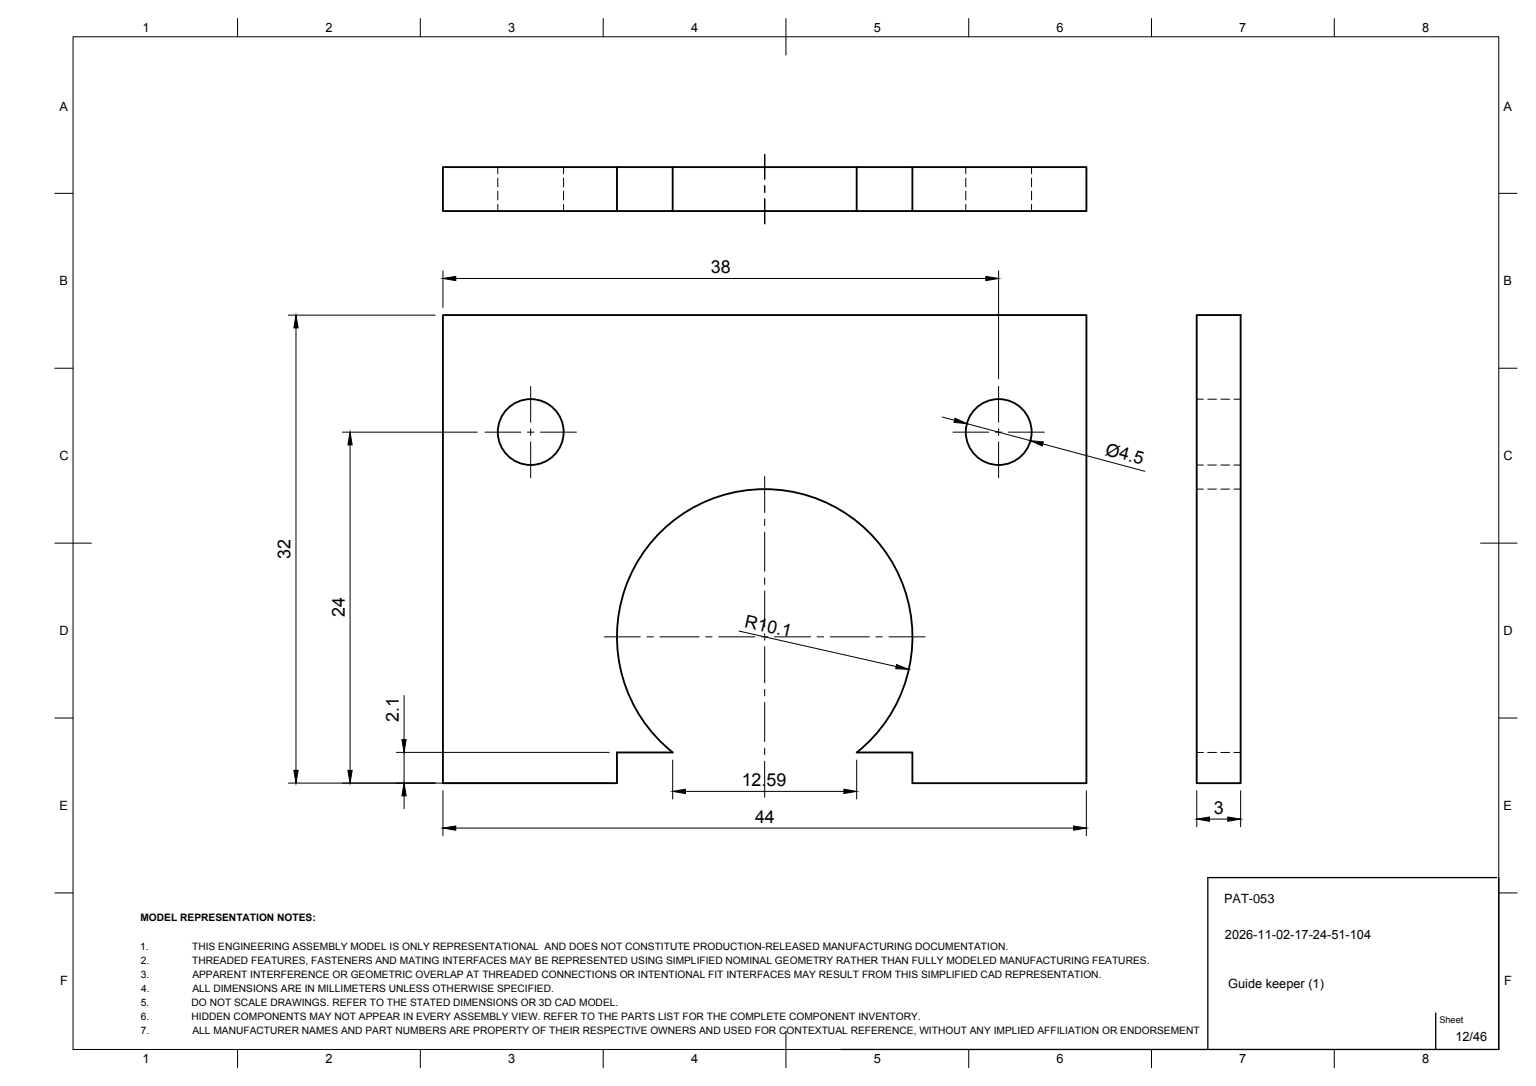
ISO-10303-21;
HEADER;
/* Generated by software containing ST-Developer
 * from STEP Tools, Inc. (www.steptools.com) 
 */

FILE_DESCRIPTION(
/* description */ ('Hand-operated arbor press'),
/* implementation_level */ '2;1');

FILE_NAME(
/* name */ 'Guide keeper (1).step',
/* time_stamp */ '2026-10-28T03:25:25-07:00',
/* author */ (''),
/* organization */ (''),
/* preprocessor_version */ 'ST-DEVELOPER v20.2',
/* originating_system */ 'Autodesk Translation Framework v15.17.0.0',
/* authorisation */ '');

FILE_SCHEMA (('AUTOMOTIVE_DESIGN { 1 0 10303 214 3 1 1 }'));
ENDSEC;

DATA;
#10=MECHANICAL_DESIGN_GEOMETRIC_PRESENTATION_REPRESENTATION('',(#593),#32751);
#509=SHAPE_REPRESENTATION_RELATIONSHIP('SRR','None',#32938,#551);
#551=ADVANCED_BREP_SHAPE_REPRESENTATION('',(#642),#32712);
#593=STYLED_ITEM('',(#33235),#642);
#642=MANIFOLD_SOLID_BREP('Body1',#12490);
#719=FACE_BOUND('',#2125,.T.);
#720=FACE_BOUND('',#2126,.T.);
#721=FACE_BOUND('',#2132,.T.);
#722=FACE_BOUND('',#2133,.T.);
#919=PLANE('',#13184);
#920=PLANE('',#13185);
#921=PLANE('',#13186);
#922=PLANE('',#13187);
#923=PLANE('',#13188);
#924=PLANE('',#13189);
#925=PLANE('',#13190);
#926=PLANE('',#13194);
#927=PLANE('',#13195);
#928=PLANE('',#13196);
#929=PLANE('',#13197);
#1396=FACE_OUTER_BOUND('',#2116,.T.);
#1397=FACE_OUTER_BOUND('',#2117,.T.);
#1398=FACE_OUTER_BOUND('',#2118,.T.);
#1399=FACE_OUTER_BOUND('',#2119,.T.);
#1400=FACE_OUTER_BOUND('',#2120,.T.);
#1401=FACE_OUTER_BOUND('',#2121,.T.);
#1402=FACE_OUTER_BOUND('',#2122,.T.);
#1403=FACE_OUTER_BOUND('',#2123,.T.);
#1404=FACE_OUTER_BOUND('',#2124,.T.);
#1405=FACE_OUTER_BOUND('',#2127,.T.);
#1406=FACE_OUTER_BOUND('',#2128,.T.);
#1407=FACE_OUTER_BOUND('',#2129,.T.);
#1408=FACE_OUTER_BOUND('',#2130,.T.);
#1409=FACE_OUTER_BOUND('',#2131,.T.);
#2116=EDGE_LOOP('',(#8816,#8817,#8818,#8819));
#2117=EDGE_LOOP('',(#8820,#8821,#8822,#8823));
#2118=EDGE_LOOP('',(#8824,#8825,#8826,#8827));
#2119=EDGE_LOOP('',(#8828,#8829,#8830,#8831));
#2120=EDGE_LOOP('',(#8832,#8833,#8834,#8835));
#2121=EDGE_LOOP('',(#8836,#8837,#8838,#8839));
#2122=EDGE_LOOP('',(#8840,#8841,#8842,#8843));
#2123=EDGE_LOOP('',(#8844,#8845,#8846,#8847));
#2124=EDGE_LOOP('',(#8848,#8849,#8850,#8851,#8852,#8853,#8854,#8855,#8856,
#8857));
#2125=EDGE_LOOP('',(#8858));
#2126=EDGE_LOOP('',(#8859));
#2127=EDGE_LOOP('',(#8860,#8861,#8862,#8863));
#2128=EDGE_LOOP('',(#8864,#8865,#8866,#8867));
#2129=EDGE_LOOP('',(#8868,#8869,#8870,#8871));
#2130=EDGE_LOOP('',(#8872,#8873,#8874,#8875));
#2131=EDGE_LOOP('',(#8876,#8877,#8878,#8879,#8880,#8881,#8882,#8883,#8884,
#8885));
#2132=EDGE_LOOP('',(#8886));
#2133=EDGE_LOOP('',(#8887));
#3004=LINE('',#18165,#4175);
#3005=LINE('',#18171,#4176);
#3006=LINE('',#18176,#4177);
#3007=LINE('',#18178,#4178);
#3008=LINE('',#18180,#4179);
#3009=LINE('',#18181,#4180);
#3010=LINE('',#18185,#4181);
#3011=LINE('',#18187,#4182);
#3012=LINE('',#18189,#4183);
#3013=LINE('',#18190,#4184);
#3014=LINE('',#18193,#4185);
#3015=LINE('',#18195,#4186);
#3016=LINE('',#18196,#4187);
#3017=LINE('',#18199,#4188);
#3018=LINE('',#18201,#4189);
#3019=LINE('',#18202,#4190);
#3020=LINE('',#18205,#4191);
#3021=LINE('',#18207,#4192);
#3022=LINE('',#18208,#4193);
#3023=LINE('',#18211,#4194);
#3024=LINE('',#18213,#4195);
#3025=LINE('',#18214,#4196);
#3026=LINE('',#18218,#4197);
#3027=LINE('',#18220,#4198);
#3028=LINE('',#18221,#4199);
#3029=LINE('',#18226,#4200);
#3030=LINE('',#18227,#4201);
#3031=LINE('',#18230,#4202);
#3032=LINE('',#18231,#4203);
#3033=LINE('',#18233,#4204);
#4175=VECTOR('',#14697,0.225);
#4176=VECTOR('',#14704,0.225);
#4177=VECTOR('',#14709,1.);
#4178=VECTOR('',#14710,1.);
#4179=VECTOR('',#14711,1.);
#4180=VECTOR('',#14712,1.);
#4181=VECTOR('',#14715,1.);
#4182=VECTOR('',#14716,1.);
#4183=VECTOR('',#14717,1.);
#4184=VECTOR('',#14718,1.);
#4185=VECTOR('',#14721,1.);
#4186=VECTOR('',#14722,1.);
#4187=VECTOR('',#14723,1.);
#4188=VECTOR('',#14726,1.);
#4189=VECTOR('',#14727,1.);
#4190=VECTOR('',#14728,1.);
#4191=VECTOR('',#14731,1.);
#4192=VECTOR('',#14732,1.);
#4193=VECTOR('',#14733,1.);
#4194=VECTOR('',#14736,1.);
#4195=VECTOR('',#14737,1.);
#4196=VECTOR('',#14738,1.);
#4197=VECTOR('',#14743,1.);
#4198=VECTOR('',#14744,1.);
#4199=VECTOR('',#14745,1.);
#4200=VECTOR('',#14752,1.);
#4201=VECTOR('',#14753,1.);
#4202=VECTOR('',#14756,1.);
#4203=VECTOR('',#14757,1.);
#4204=VECTOR('',#14760,1.);
#5232=CIRCLE('',#13179,0.225);
#5233=CIRCLE('',#13180,0.225);
#5234=CIRCLE('',#13182,0.225);
#5235=CIRCLE('',#13183,0.225);
#5236=CIRCLE('',#13191,1.01);
#5237=CIRCLE('',#13193,1.01);
#5720=VERTEX_POINT('',#18162);
#5721=VERTEX_POINT('',#18164);
#5722=VERTEX_POINT('',#18168);
#5723=VERTEX_POINT('',#18170);
#5724=VERTEX_POINT('',#18174);
#5725=VERTEX_POINT('',#18175);
#5726=VERTEX_POINT('',#18177);
#5727=VERTEX_POINT('',#18179);
#5728=VERTEX_POINT('',#18183);
#5729=VERTEX_POINT('',#18184);
#5730=VERTEX_POINT('',#18186);
#5731=VERTEX_POINT('',#18188);
#5732=VERTEX_POINT('',#18192);
#5733=VERTEX_POINT('',#18194);
#5734=VERTEX_POINT('',#18198);
#5735=VERTEX_POINT('',#18200);
#5736=VERTEX_POINT('',#18204);
#5737=VERTEX_POINT('',#18206);
#5738=VERTEX_POINT('',#18210);
#5739=VERTEX_POINT('',#18212);
#5740=VERTEX_POINT('',#18217);
#5741=VERTEX_POINT('',#18219);
#5742=VERTEX_POINT('',#18225);
#5743=VERTEX_POINT('',#18229);
#6911=EDGE_CURVE('',#5720,#5720,#5232,.T.);
#6912=EDGE_CURVE('',#5720,#5721,#3004,.T.);
#6913=EDGE_CURVE('',#5721,#5721,#5233,.T.);
#6914=EDGE_CURVE('',#5722,#5722,#5234,.T.);
#6915=EDGE_CURVE('',#5722,#5723,#3005,.T.);
#6916=EDGE_CURVE('',#5723,#5723,#5235,.T.);
#6917=EDGE_CURVE('',#5724,#5725,#3006,.T.);
#6918=EDGE_CURVE('',#5724,#5726,#3007,.T.);
#6919=EDGE_CURVE('',#5727,#5726,#3008,.T.);
#6920=EDGE_CURVE('',#5725,#5727,#3009,.T.);
#6921=EDGE_CURVE('',#5728,#5729,#3010,.T.);
#6922=EDGE_CURVE('',#5730,#5728,#3011,.T.);
#6923=EDGE_CURVE('',#5731,#5730,#3012,.T.);
#6924=EDGE_CURVE('',#5729,#5731,#3013,.T.);
#6925=EDGE_CURVE('',#5732,#5728,#3014,.T.);
#6926=EDGE_CURVE('',#5733,#5732,#3015,.T.);
#6927=EDGE_CURVE('',#5730,#5733,#3016,.T.);
#6928=EDGE_CURVE('',#5734,#5724,#3017,.T.);
#6929=EDGE_CURVE('',#5735,#5734,#3018,.T.);
#6930=EDGE_CURVE('',#5726,#5735,#3019,.T.);
#6931=EDGE_CURVE('',#5736,#5727,#3020,.T.);
#6932=EDGE_CURVE('',#5737,#5736,#3021,.T.);
#6933=EDGE_CURVE('',#5737,#5725,#3022,.T.);
#6934=EDGE_CURVE('',#5731,#5738,#3023,.T.);
#6935=EDGE_CURVE('',#5738,#5739,#3024,.T.);
#6936=EDGE_CURVE('',#5729,#5739,#3025,.T.);
#6937=EDGE_CURVE('',#5735,#5732,#5236,.T.);
#6938=EDGE_CURVE('',#5739,#5740,#3026,.T.);
#6939=EDGE_CURVE('',#5740,#5741,#3027,.T.);
#6940=EDGE_CURVE('',#5741,#5736,#3028,.T.);
#6941=EDGE_CURVE('',#5733,#5734,#5237,.T.);
#6942=EDGE_CURVE('',#5742,#5737,#3029,.T.);
#6943=EDGE_CURVE('',#5742,#5741,#3030,.T.);
#6944=EDGE_CURVE('',#5743,#5742,#3031,.T.);
#6945=EDGE_CURVE('',#5743,#5740,#3032,.T.);
#6946=EDGE_CURVE('',#5738,#5743,#3033,.T.);
#8816=ORIENTED_EDGE('',*,*,#6911,.F.);
#8817=ORIENTED_EDGE('',*,*,#6912,.T.);
#8818=ORIENTED_EDGE('',*,*,#6913,.F.);
#8819=ORIENTED_EDGE('',*,*,#6912,.F.);
#8820=ORIENTED_EDGE('',*,*,#6914,.F.);
#8821=ORIENTED_EDGE('',*,*,#6915,.T.);
#8822=ORIENTED_EDGE('',*,*,#6916,.F.);
#8823=ORIENTED_EDGE('',*,*,#6915,.F.);
#8824=ORIENTED_EDGE('',*,*,#6917,.F.);
#8825=ORIENTED_EDGE('',*,*,#6918,.T.);
#8826=ORIENTED_EDGE('',*,*,#6919,.F.);
#8827=ORIENTED_EDGE('',*,*,#6920,.F.);
#8828=ORIENTED_EDGE('',*,*,#6921,.F.);
#8829=ORIENTED_EDGE('',*,*,#6922,.F.);
#8830=ORIENTED_EDGE('',*,*,#6923,.F.);
#8831=ORIENTED_EDGE('',*,*,#6924,.F.);
#8832=ORIENTED_EDGE('',*,*,#6925,.F.);
#8833=ORIENTED_EDGE('',*,*,#6926,.F.);
#8834=ORIENTED_EDGE('',*,*,#6927,.F.);
#8835=ORIENTED_EDGE('',*,*,#6922,.T.);
#8836=ORIENTED_EDGE('',*,*,#6928,.F.);
#8837=ORIENTED_EDGE('',*,*,#6929,.F.);
#8838=ORIENTED_EDGE('',*,*,#6930,.F.);
#8839=ORIENTED_EDGE('',*,*,#6918,.F.);
#8840=ORIENTED_EDGE('',*,*,#6920,.T.);
#8841=ORIENTED_EDGE('',*,*,#6931,.F.);
#8842=ORIENTED_EDGE('',*,*,#6932,.F.);
#8843=ORIENTED_EDGE('',*,*,#6933,.T.);
#8844=ORIENTED_EDGE('',*,*,#6924,.T.);
#8845=ORIENTED_EDGE('',*,*,#6934,.T.);
#8846=ORIENTED_EDGE('',*,*,#6935,.T.);
#8847=ORIENTED_EDGE('',*,*,#6936,.F.);
#8848=ORIENTED_EDGE('',*,*,#6919,.T.);
#8849=ORIENTED_EDGE('',*,*,#6930,.T.);
#8850=ORIENTED_EDGE('',*,*,#6937,.T.);
#8851=ORIENTED_EDGE('',*,*,#6925,.T.);
#8852=ORIENTED_EDGE('',*,*,#6921,.T.);
#8853=ORIENTED_EDGE('',*,*,#6936,.T.);
#8854=ORIENTED_EDGE('',*,*,#6938,.T.);
#8855=ORIENTED_EDGE('',*,*,#6939,.T.);
#8856=ORIENTED_EDGE('',*,*,#6940,.T.);
#8857=ORIENTED_EDGE('',*,*,#6931,.T.);
#8858=ORIENTED_EDGE('',*,*,#6913,.T.);
#8859=ORIENTED_EDGE('',*,*,#6916,.T.);
#8860=ORIENTED_EDGE('',*,*,#6929,.T.);
#8861=ORIENTED_EDGE('',*,*,#6941,.F.);
#8862=ORIENTED_EDGE('',*,*,#6926,.T.);
#8863=ORIENTED_EDGE('',*,*,#6937,.F.);
#8864=ORIENTED_EDGE('',*,*,#6942,.T.);
#8865=ORIENTED_EDGE('',*,*,#6932,.T.);
#8866=ORIENTED_EDGE('',*,*,#6940,.F.);
#8867=ORIENTED_EDGE('',*,*,#6943,.F.);
#8868=ORIENTED_EDGE('',*,*,#6944,.T.);
#8869=ORIENTED_EDGE('',*,*,#6943,.T.);
#8870=ORIENTED_EDGE('',*,*,#6939,.F.);
#8871=ORIENTED_EDGE('',*,*,#6945,.F.);
#8872=ORIENTED_EDGE('',*,*,#6946,.T.);
#8873=ORIENTED_EDGE('',*,*,#6945,.T.);
#8874=ORIENTED_EDGE('',*,*,#6938,.F.);
#8875=ORIENTED_EDGE('',*,*,#6935,.F.);
#8876=ORIENTED_EDGE('',*,*,#6917,.T.);
#8877=ORIENTED_EDGE('',*,*,#6933,.F.);
#8878=ORIENTED_EDGE('',*,*,#6942,.F.);
#8879=ORIENTED_EDGE('',*,*,#6944,.F.);
#8880=ORIENTED_EDGE('',*,*,#6946,.F.);
#8881=ORIENTED_EDGE('',*,*,#6934,.F.);
#8882=ORIENTED_EDGE('',*,*,#6923,.T.);
#8883=ORIENTED_EDGE('',*,*,#6927,.T.);
#8884=ORIENTED_EDGE('',*,*,#6941,.T.);
#8885=ORIENTED_EDGE('',*,*,#6928,.T.);
#8886=ORIENTED_EDGE('',*,*,#6911,.T.);
#8887=ORIENTED_EDGE('',*,*,#6914,.T.);
#11675=CYLINDRICAL_SURFACE('',#13178,0.225);
#11676=CYLINDRICAL_SURFACE('',#13181,0.225);
#11677=CYLINDRICAL_SURFACE('',#13192,1.01);
#11905=ADVANCED_FACE('',(#1396),#11675,.F.);
#11906=ADVANCED_FACE('',(#1397),#11676,.F.);
#11907=ADVANCED_FACE('',(#1398),#919,.F.);
#11908=ADVANCED_FACE('',(#1399),#920,.F.);
#11909=ADVANCED_FACE('',(#1400),#921,.F.);
#11910=ADVANCED_FACE('',(#1401),#922,.F.);
#11911=ADVANCED_FACE('',(#1402),#923,.T.);
#11912=ADVANCED_FACE('',(#1403),#924,.T.);
#11913=ADVANCED_FACE('',(#1404,#719,#720),#925,.T.);
#11914=ADVANCED_FACE('',(#1405),#11677,.F.);
#11915=ADVANCED_FACE('',(#1406),#926,.T.);
#11916=ADVANCED_FACE('',(#1407),#927,.T.);
#11917=ADVANCED_FACE('',(#1408),#928,.T.);
#11918=ADVANCED_FACE('',(#1409,#721,#722),#929,.F.);
#12490=CLOSED_SHELL('',(#11905,#11906,#11907,#11908,#11909,#11910,#11911,
#11912,#11913,#11914,#11915,#11916,#11917,#11918));
#13177=AXIS2_PLACEMENT_3D('',#18160,#14691,#14692);
#13178=AXIS2_PLACEMENT_3D('',#18161,#14693,#14694);
#13179=AXIS2_PLACEMENT_3D('',#18163,#14695,#14696);
#13180=AXIS2_PLACEMENT_3D('',#18166,#14698,#14699);
#13181=AXIS2_PLACEMENT_3D('',#18167,#14700,#14701);
#13182=AXIS2_PLACEMENT_3D('',#18169,#14702,#14703);
#13183=AXIS2_PLACEMENT_3D('',#18172,#14705,#14706);
#13184=AXIS2_PLACEMENT_3D('',#18173,#14707,#14708);
#13185=AXIS2_PLACEMENT_3D('',#18182,#14713,#14714);
#13186=AXIS2_PLACEMENT_3D('',#18191,#14719,#14720);
#13187=AXIS2_PLACEMENT_3D('',#18197,#14724,#14725);
#13188=AXIS2_PLACEMENT_3D('',#18203,#14729,#14730);
#13189=AXIS2_PLACEMENT_3D('',#18209,#14734,#14735);
#13190=AXIS2_PLACEMENT_3D('',#18215,#14739,#14740);
#13191=AXIS2_PLACEMENT_3D('',#18216,#14741,#14742);
#13192=AXIS2_PLACEMENT_3D('',#18222,#14746,#14747);
#13193=AXIS2_PLACEMENT_3D('',#18223,#14748,#14749);
#13194=AXIS2_PLACEMENT_3D('',#18224,#14750,#14751);
#13195=AXIS2_PLACEMENT_3D('',#18228,#14754,#14755);
#13196=AXIS2_PLACEMENT_3D('',#18232,#14758,#14759);
#13197=AXIS2_PLACEMENT_3D('',#18234,#14761,#14762);
#14691=DIRECTION('axis',(0.,0.,1.));
#14692=DIRECTION('refdir',(1.,0.,0.));
#14693=DIRECTION('center_axis',(0.,0.,1.));
#14694=DIRECTION('ref_axis',(1.,0.,0.));
#14695=DIRECTION('center_axis',(0.,0.,1.));
#14696=DIRECTION('ref_axis',(1.,0.,0.));
#14697=DIRECTION('',(0.,0.,1.));
#14698=DIRECTION('center_axis',(0.,0.,-1.));
#14699=DIRECTION('ref_axis',(1.,0.,0.));
#14700=DIRECTION('center_axis',(0.,0.,1.));
#14701=DIRECTION('ref_axis',(1.,0.,0.));
#14702=DIRECTION('center_axis',(0.,0.,1.));
#14703=DIRECTION('ref_axis',(1.,0.,0.));
#14704=DIRECTION('',(0.,0.,1.));
#14705=DIRECTION('center_axis',(0.,0.,-1.));
#14706=DIRECTION('ref_axis',(1.,0.,0.));
#14707=DIRECTION('center_axis',(0.,1.,0.));
#14708=DIRECTION('ref_axis',(-1.,0.,0.));
#14709=DIRECTION('',(-1.,0.,0.));
#14710=DIRECTION('',(0.,0.,1.));
#14711=DIRECTION('',(1.,0.,0.));
#14712=DIRECTION('',(0.,0.,1.));
#14713=DIRECTION('center_axis',(0.,-1.,0.));
#14714=DIRECTION('ref_axis',(1.,0.,0.));
#14715=DIRECTION('',(-1.,0.,0.));
#14716=DIRECTION('',(0.,0.,1.));
#14717=DIRECTION('',(1.,0.,0.));
#14718=DIRECTION('',(0.,0.,-1.));
#14719=DIRECTION('center_axis',(1.,0.,0.));
#14720=DIRECTION('ref_axis',(0.,1.,0.));
#14721=DIRECTION('',(0.,-1.,0.));
#14722=DIRECTION('',(0.,0.,1.));
#14723=DIRECTION('',(0.,1.,0.));
#14724=DIRECTION('center_axis',(1.,0.,0.));
#14725=DIRECTION('ref_axis',(0.,1.,0.));
#14726=DIRECTION('',(0.,1.,0.));
#14727=DIRECTION('',(0.,0.,-1.));
#14728=DIRECTION('',(0.,-1.,0.));
#14729=DIRECTION('center_axis',(-1.,0.,0.));
#14730=DIRECTION('ref_axis',(0.,-1.,0.));
#14731=DIRECTION('',(0.,-1.,0.));
#14732=DIRECTION('',(0.,0.,1.));
#14733=DIRECTION('',(0.,-1.,0.));
#14734=DIRECTION('center_axis',(-1.,0.,0.));
#14735=DIRECTION('ref_axis',(0.,-1.,0.));
#14736=DIRECTION('',(0.,-1.,0.));
#14737=DIRECTION('',(0.,0.,1.));
#14738=DIRECTION('',(0.,-1.,0.));
#14739=DIRECTION('center_axis',(0.,0.,1.));
#14740=DIRECTION('ref_axis',(1.,0.,0.));
#14741=DIRECTION('center_axis',(0.,0.,-1.));
#14742=DIRECTION('ref_axis',(1.,0.,0.));
#14743=DIRECTION('',(1.,0.,0.));
#14744=DIRECTION('',(0.,1.,0.));
#14745=DIRECTION('',(-1.,0.,0.));
#14746=DIRECTION('center_axis',(0.,0.,1.));
#14747=DIRECTION('ref_axis',(1.,0.,0.));
#14748=DIRECTION('center_axis',(0.,0.,1.));
#14749=DIRECTION('ref_axis',(1.,0.,0.));
#14750=DIRECTION('center_axis',(0.,1.,0.));
#14751=DIRECTION('ref_axis',(-1.,0.,0.));
#14752=DIRECTION('',(-1.,0.,0.));
#14753=DIRECTION('',(0.,0.,1.));
#14754=DIRECTION('center_axis',(1.,0.,0.));
#14755=DIRECTION('ref_axis',(0.,1.,0.));
#14756=DIRECTION('',(0.,1.,0.));
#14757=DIRECTION('',(0.,0.,1.));
#14758=DIRECTION('center_axis',(0.,-1.,0.));
#14759=DIRECTION('ref_axis',(1.,0.,0.));
#14760=DIRECTION('',(1.,0.,0.));
#14761=DIRECTION('center_axis',(0.,0.,1.));
#14762=DIRECTION('ref_axis',(1.,0.,0.));
#18160=CARTESIAN_POINT('',(0.,0.,0.));
#18161=CARTESIAN_POINT('Origin',(2.4,-1.6,25.2));
#18162=CARTESIAN_POINT('',(2.175,-1.6,25.3));
#18163=CARTESIAN_POINT('Origin',(2.4,-1.6,25.3));
#18164=CARTESIAN_POINT('',(2.175,-1.6,25.6));
#18165=CARTESIAN_POINT('',(2.175,-1.6,25.2));
#18166=CARTESIAN_POINT('Origin',(2.4,-1.6,25.6));
#18167=CARTESIAN_POINT('Origin',(2.4,1.6,25.2));
#18168=CARTESIAN_POINT('',(2.175,1.6,25.3));
#18169=CARTESIAN_POINT('Origin',(2.4,1.6,25.3));
#18170=CARTESIAN_POINT('',(2.175,1.6,25.6));
#18171=CARTESIAN_POINT('',(2.175,1.6,25.2));
#18172=CARTESIAN_POINT('Origin',(2.4,1.6,25.6));
#18173=CARTESIAN_POINT('Origin',(0.21,1.01,25.2));
#18174=CARTESIAN_POINT('',(0.21,1.01,25.3));
#18175=CARTESIAN_POINT('',(0.,1.01,25.3));
#18176=CARTESIAN_POINT('',(0.905,1.01,25.3));
#18177=CARTESIAN_POINT('',(0.21,1.01,25.6));
#18178=CARTESIAN_POINT('',(0.21,1.01,25.2));
#18179=CARTESIAN_POINT('',(0.,1.01,25.6));
#18180=CARTESIAN_POINT('',(0.905,1.01,25.6));
#18181=CARTESIAN_POINT('',(0.,1.01,25.25));
#18182=CARTESIAN_POINT('Origin',(-0.1,-1.01,25.2));
#18183=CARTESIAN_POINT('',(0.21,-1.01,25.6));
#18184=CARTESIAN_POINT('',(0.,-1.01,25.6));
#18185=CARTESIAN_POINT('',(0.75,-1.01,25.6));
#18186=CARTESIAN_POINT('',(0.21,-1.01,25.3));
#18187=CARTESIAN_POINT('',(0.21,-1.01,25.2));
#18188=CARTESIAN_POINT('',(0.,-1.01,25.3));
#18189=CARTESIAN_POINT('',(0.75,-1.01,25.3));
#18190=CARTESIAN_POINT('',(0.,-1.01,25.25));
#18191=CARTESIAN_POINT('Origin',(0.21,-1.01,25.2));
#18192=CARTESIAN_POINT('',(0.21,-0.629285308902091,25.6));
#18193=CARTESIAN_POINT('',(0.21,-0.505,25.6));
#18194=CARTESIAN_POINT('',(0.21,-0.629285308902091,25.3));
#18195=CARTESIAN_POINT('',(0.21,-0.629285308902091,25.2));
#18196=CARTESIAN_POINT('',(0.21,-0.505,25.3));
#18197=CARTESIAN_POINT('Origin',(0.21,-1.01,25.2));
#18198=CARTESIAN_POINT('',(0.21,0.629285308902091,25.3));
#18199=CARTESIAN_POINT('',(0.21,-0.505,25.3));
#18200=CARTESIAN_POINT('',(0.21,0.629285308902091,25.6));
#18201=CARTESIAN_POINT('',(0.21,0.629285308902091,25.2));
#18202=CARTESIAN_POINT('',(0.21,-0.505,25.6));
#18203=CARTESIAN_POINT('Origin',(0.,2.2,25.3));
#18204=CARTESIAN_POINT('',(0.,2.2,25.6));
#18205=CARTESIAN_POINT('',(0.,2.2,25.6));
#18206=CARTESIAN_POINT('',(0.,2.2,25.3));
#18207=CARTESIAN_POINT('',(0.,2.2,25.3));
#18208=CARTESIAN_POINT('',(0.,2.2,25.3));
#18209=CARTESIAN_POINT('Origin',(0.,2.2,25.3));
#18210=CARTESIAN_POINT('',(0.,-2.2,25.3));
#18211=CARTESIAN_POINT('',(0.,2.2,25.3));
#18212=CARTESIAN_POINT('',(0.,-2.2,25.6));
#18213=CARTESIAN_POINT('',(0.,-2.2,25.3));
#18214=CARTESIAN_POINT('',(0.,2.2,25.6));
#18215=CARTESIAN_POINT('Origin',(1.6,0.,25.6));
#18216=CARTESIAN_POINT('Origin',(1.,0.,25.6));
#18217=CARTESIAN_POINT('',(3.2,-2.2,25.6));
#18218=CARTESIAN_POINT('',(0.,-2.2,25.6));
#18219=CARTESIAN_POINT('',(3.2,2.2,25.6));
#18220=CARTESIAN_POINT('',(3.2,-2.2,25.6));
#18221=CARTESIAN_POINT('',(3.2,2.2,25.6));
#18222=CARTESIAN_POINT('Origin',(1.,0.,25.2));
#18223=CARTESIAN_POINT('Origin',(1.,0.,25.3));
#18224=CARTESIAN_POINT('Origin',(3.2,2.2,25.3));
#18225=CARTESIAN_POINT('',(3.2,2.2,25.3));
#18226=CARTESIAN_POINT('',(3.2,2.2,25.3));
#18227=CARTESIAN_POINT('',(3.2,2.2,25.3));
#18228=CARTESIAN_POINT('Origin',(3.2,-2.2,25.3));
#18229=CARTESIAN_POINT('',(3.2,-2.2,25.3));
#18230=CARTESIAN_POINT('',(3.2,-2.2,25.3));
#18231=CARTESIAN_POINT('',(3.2,-2.2,25.3));
#18232=CARTESIAN_POINT('Origin',(0.,-2.2,25.3));
#18233=CARTESIAN_POINT('',(0.,-2.2,25.3));
#18234=CARTESIAN_POINT('Origin',(1.6,0.,25.3));
#32663=UNCERTAINTY_MEASURE_WITH_UNIT(LENGTH_MEASURE(0.001),#32752,
'DISTANCE_ACCURACY_VALUE',
'Maximum model space distance between geometric entities at asserted c
onnectivities');
#32702=UNCERTAINTY_MEASURE_WITH_UNIT(LENGTH_MEASURE(0.001),#32752,
'DISTANCE_ACCURACY_VALUE',
'Maximum model space distance between geometric entities at asserted c
onnectivities');
#32712=(
GEOMETRIC_REPRESENTATION_CONTEXT(3)
GLOBAL_UNCERTAINTY_ASSIGNED_CONTEXT((#32663))
GLOBAL_UNIT_ASSIGNED_CONTEXT((#32752,#32754,#32755))
REPRESENTATION_CONTEXT('','3D')
);
#32751=(
GEOMETRIC_REPRESENTATION_CONTEXT(3)
GLOBAL_UNCERTAINTY_ASSIGNED_CONTEXT((#32702))
GLOBAL_UNIT_ASSIGNED_CONTEXT((#32752,#32754,#32755))
REPRESENTATION_CONTEXT('','3D')
);
#32752=(
LENGTH_UNIT()
NAMED_UNIT(*)
SI_UNIT(.CENTI.,.METRE.)
);
#32754=(
NAMED_UNIT(*)
PLANE_ANGLE_UNIT()
SI_UNIT($,.RADIAN.)
);
#32755=(
NAMED_UNIT(*)
SI_UNIT($,.STERADIAN.)
SOLID_ANGLE_UNIT()
);
#32765=SHAPE_DEFINITION_REPRESENTATION(#32813,#32938);
#32813=PRODUCT_DEFINITION_SHAPE('',$,#32987);
#32938=SHAPE_REPRESENTATION('',(#13177),#32712);
#32977=PRODUCT_DEFINITION_CONTEXT('part definition',#33123,'design');
#32987=PRODUCT_DEFINITION('Guide keeper (1)','Guide keeper (1)',#33035,#32977);
#33035=PRODUCT_DEFINITION_FORMATION('',$,#33134);
#33123=APPLICATION_CONTEXT(
'Core Data for Automotive Mechanical Design Process');
#33124=PRODUCT_CONTEXT('part definition',#33123,'mechanical');
#33134=PRODUCT('Guide keeper (1)','Guide keeper (1)','Guide keeper (1)',(#33124));
#33229=COLOUR_RGB('Sky Blue',0.24,0.69,0.87);
#33230=FILL_AREA_STYLE_COLOUR('',#33229);
#33231=FILL_AREA_STYLE('',(#33230));
#33232=SURFACE_STYLE_FILL_AREA(#33231);
#33233=SURFACE_SIDE_STYLE('',(#33232));
#33234=SURFACE_STYLE_USAGE(.BOTH.,#33233);
#33235=PRESENTATION_STYLE_ASSIGNMENT((#33234));
ENDSEC;
END-ISO-10303-21;
